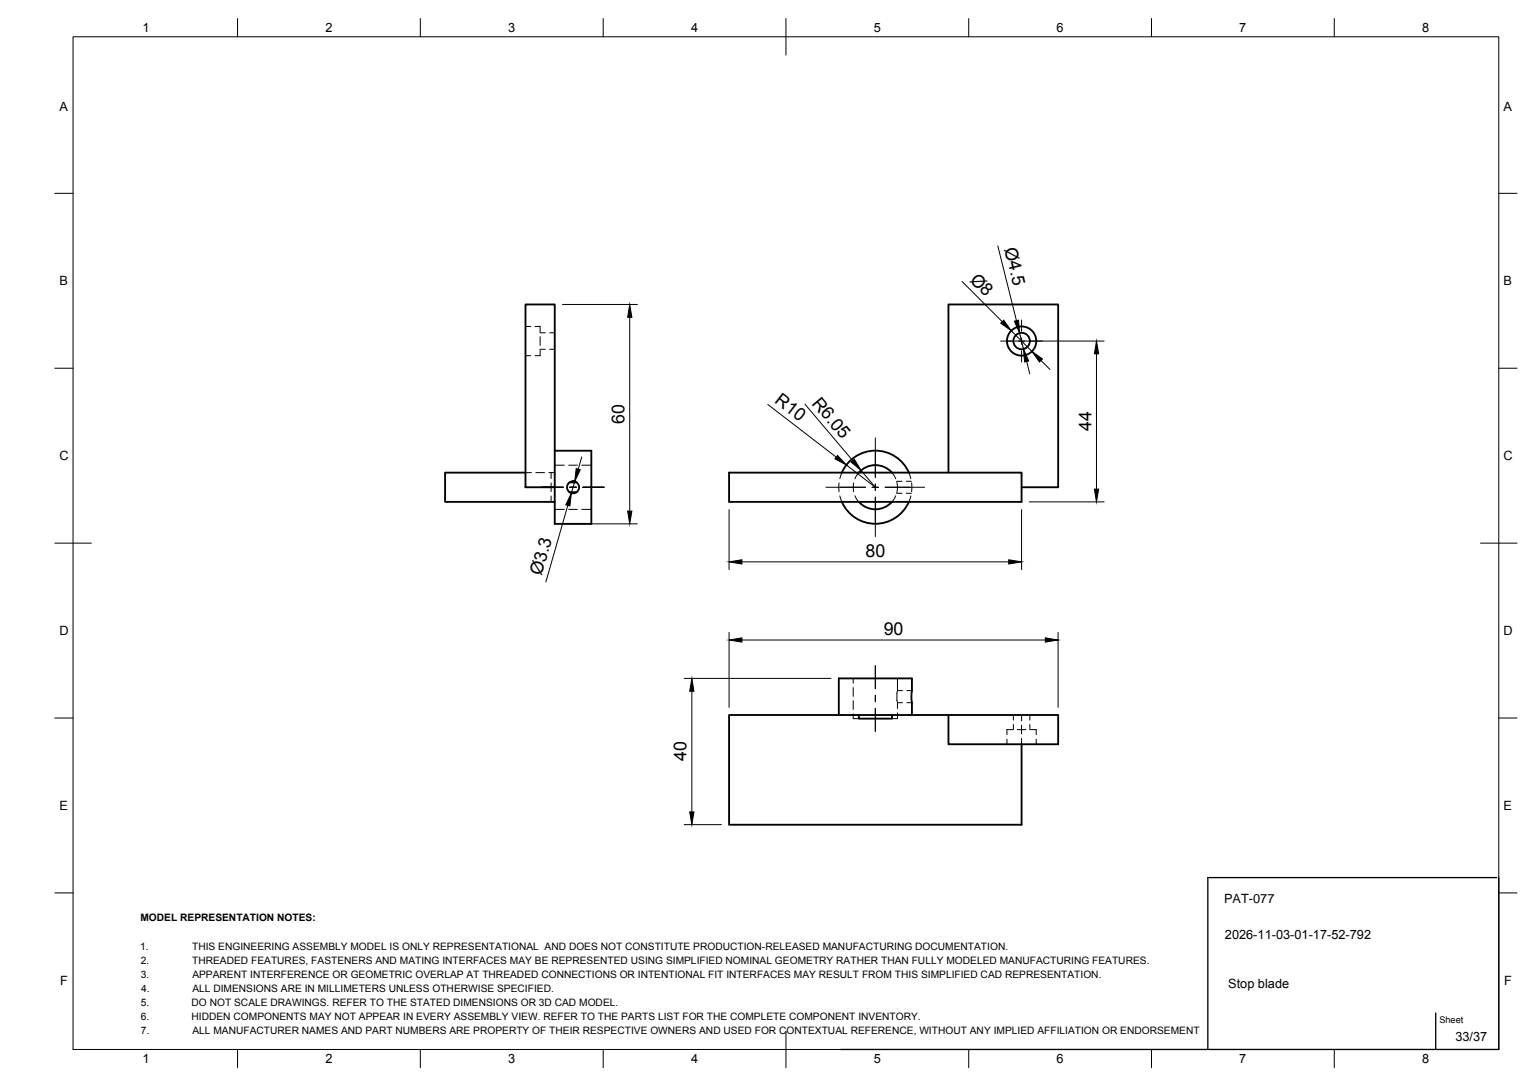
ISO-10303-21;
HEADER;
/* Generated by software containing ST-Developer
 * from STEP Tools, Inc. (www.steptools.com) 
 */

FILE_DESCRIPTION(
/* description */ ('Pallet stop with pneumatic fitting'),
/* implementation_level */ '2;1');

FILE_NAME(
/* name */ 'Stop blade.step',
/* time_stamp */ '2026-10-27T10:51:41-07:00',
/* author */ (''),
/* organization */ (''),
/* preprocessor_version */ 'ST-DEVELOPER v20.2',
/* originating_system */ 'Autodesk Translation Framework v15.17.0.0',
/* authorisation */ '');

FILE_SCHEMA (('AUTOMOTIVE_DESIGN { 1 0 10303 214 3 1 1 }'));
ENDSEC;

DATA;
#10=MECHANICAL_DESIGN_GEOMETRIC_PRESENTATION_REPRESENTATION('',(#382),#10265);
#287=B_SPLINE_CURVE_WITH_KNOTS('',3,(#9812,#9813,#9814,#9815,#9816,#9817,
#9818,#9819,#9820,#9821,#9822,#9823,#9824,#9825),.UNSPECIFIED.,.F.,.F.,
(4,2,2,2,2,2,4),(0.598759573717651,0.624973342427789,0.687463163426141,
0.749952984424493,0.812442805422845,0.874932626421197,0.901146395131335),
 .UNSPECIFIED.);
#288=B_SPLINE_CURVE_WITH_KNOTS('',3,(#9829,#9830,#9831,#9832,#9833,#9834,
#9835,#9836),.UNSPECIFIED.,.F.,.F.,(4,2,2,4),(0.249984328141498,0.31247414913985,
0.374963970138202,0.401177738848337),.UNSPECIFIED.);
#289=B_SPLINE_CURVE_WITH_KNOTS('',3,(#9840,#9841,#9842,#9843,#9844,#9845,
#9846,#9847,#9848,#9849,#9850,#9851,#9852,#9853,#9854,#9855,#9856,#9857,
#9858,#9859,#9860,#9861,#9862,#9863,#9864,#9865),.UNSPECIFIED.,.F.,.F.,
(4,2,2,2,2,2,2,2,2,2,2,2,4),(0.,0.0622766332261793,0.124553266452359,0.186828302721277,
0.249103338990195,0.311378375259114,0.373653411528032,0.435930044754212,
0.498206677980391,0.56048331120657,0.62275994443275,0.685034980701668,0.747310016970586),
 .UNSPECIFIED.);
#290=B_SPLINE_CURVE_WITH_KNOTS('',3,(#9866,#9867,#9868,#9869,#9870,#9871,
#9872,#9873,#9874,#9875),.UNSPECIFIED.,.F.,.F.,(4,2,2,2,4),(0.747310016970586,
0.809585053239505,0.871860089508423,0.934136722734602,0.996413355960782),
 .UNSPECIFIED.);
#291=B_SPLINE_CURVE_WITH_KNOTS('',3,(#9876,#9877,#9878,#9879,#9880,#9881,
#9882,#9883),.UNSPECIFIED.,.F.,.F.,(4,2,2,4),(0.0987909174346565,0.125004686144793,
0.187494507143146,0.249984328141498),.UNSPECIFIED.);
#318=SHAPE_REPRESENTATION_RELATIONSHIP('SRR','None',#10434,#350);
#350=ADVANCED_BREP_SHAPE_REPRESENTATION('',(#413),#10258);
#382=STYLED_ITEM('',(#10641),#413);
#413=MANIFOLD_SOLID_BREP('Body1',#5071);
#529=FACE_BOUND('',#1401,.T.);
#530=FACE_BOUND('',#1408,.T.);
#531=FACE_BOUND('',#1416,.T.);
#532=FACE_BOUND('',#1421,.T.);
#533=FACE_BOUND('',#1423,.T.);
#534=FACE_BOUND('',#1426,.T.);
#685=PLANE('',#5905);
#686=PLANE('',#5909);
#687=PLANE('',#5910);
#688=PLANE('',#5911);
#689=PLANE('',#5912);
#690=PLANE('',#5913);
#691=PLANE('',#5914);
#692=PLANE('',#5915);
#693=PLANE('',#5916);
#694=PLANE('',#5920);
#695=PLANE('',#5921);
#696=PLANE('',#5929);
#697=PLANE('',#5930);
#698=PLANE('',#5932);
#699=PLANE('',#5939);
#700=PLANE('',#5940);
#701=PLANE('',#5941);
#702=PLANE('',#5942);
#703=PLANE('',#5943);
#975=FACE_OUTER_BOUND('',#1399,.T.);
#976=FACE_OUTER_BOUND('',#1400,.T.);
#977=FACE_OUTER_BOUND('',#1402,.T.);
#978=FACE_OUTER_BOUND('',#1403,.T.);
#979=FACE_OUTER_BOUND('',#1404,.T.);
#980=FACE_OUTER_BOUND('',#1405,.T.);
#981=FACE_OUTER_BOUND('',#1406,.T.);
#982=FACE_OUTER_BOUND('',#1407,.T.);
#983=FACE_OUTER_BOUND('',#1409,.T.);
#984=FACE_OUTER_BOUND('',#1410,.T.);
#985=FACE_OUTER_BOUND('',#1411,.T.);
#986=FACE_OUTER_BOUND('',#1412,.T.);
#987=FACE_OUTER_BOUND('',#1413,.T.);
#988=FACE_OUTER_BOUND('',#1414,.T.);
#989=FACE_OUTER_BOUND('',#1415,.T.);
#990=FACE_OUTER_BOUND('',#1417,.T.);
#991=FACE_OUTER_BOUND('',#1418,.T.);
#992=FACE_OUTER_BOUND('',#1419,.T.);
#993=FACE_OUTER_BOUND('',#1420,.T.);
#994=FACE_OUTER_BOUND('',#1422,.T.);
#995=FACE_OUTER_BOUND('',#1424,.T.);
#996=FACE_OUTER_BOUND('',#1425,.T.);
#997=FACE_OUTER_BOUND('',#1427,.T.);
#998=FACE_OUTER_BOUND('',#1428,.T.);
#1399=EDGE_LOOP('',(#4310,#4311,#4312,#4313));
#1400=EDGE_LOOP('',(#4314));
#1401=EDGE_LOOP('',(#4315));
#1402=EDGE_LOOP('',(#4316,#4317,#4318,#4319));
#1403=EDGE_LOOP('',(#4320,#4321,#4322,#4323));
#1404=EDGE_LOOP('',(#4324,#4325,#4326,#4327));
#1405=EDGE_LOOP('',(#4328,#4329,#4330,#4331));
#1406=EDGE_LOOP('',(#4332,#4333,#4334,#4335));
#1407=EDGE_LOOP('',(#4336,#4337,#4338,#4339,#4340,#4341));
#1408=EDGE_LOOP('',(#4342));
#1409=EDGE_LOOP('',(#4343,#4344,#4345,#4346,#4347,#4348));
#1410=EDGE_LOOP('',(#4349,#4350,#4351,#4352,#4353,#4354,#4355,#4356,#4357,
#4358,#4359,#4360));
#1411=EDGE_LOOP('',(#4361,#4362));
#1412=EDGE_LOOP('',(#4363,#4364,#4365,#4366,#4367,#4368,#4369,#4370,#4371));
#1413=EDGE_LOOP('',(#4372,#4373));
#1414=EDGE_LOOP('',(#4374,#4375,#4376,#4377,#4378));
#1415=EDGE_LOOP('',(#4379,#4380,#4381,#4382,#4383,#4384,#4385,#4386,#4387,
#4388,#4389,#4390));
#1416=EDGE_LOOP('',(#4391,#4392,#4393,#4394,#4395));
#1417=EDGE_LOOP('',(#4396,#4397,#4398,#4399,#4400,#4401,#4402,#4403,#4404,
#4405));
#1418=EDGE_LOOP('',(#4406,#4407,#4408,#4409));
#1419=EDGE_LOOP('',(#4410,#4411,#4412,#4413));
#1420=EDGE_LOOP('',(#4414,#4415,#4416,#4417,#4418,#4419,#4420,#4421));
#1421=EDGE_LOOP('',(#4422,#4423));
#1422=EDGE_LOOP('',(#4424));
#1423=EDGE_LOOP('',(#4425));
#1424=EDGE_LOOP('',(#4426,#4427,#4428,#4429,#4430));
#1425=EDGE_LOOP('',(#4431,#4432,#4433,#4434,#4435,#4436,#4437,#4438));
#1426=EDGE_LOOP('',(#4439));
#1427=EDGE_LOOP('',(#4440,#4441,#4442,#4443));
#1428=EDGE_LOOP('',(#4444,#4445,#4446,#4447));
#1724=LINE('',#9739,#2059);
#1725=LINE('',#9747,#2060);
#1726=LINE('',#9751,#2061);
#1727=LINE('',#9753,#2062);
#1728=LINE('',#9755,#2063);
#1729=LINE('',#9756,#2064);
#1730=LINE('',#9759,#2065);
#1731=LINE('',#9761,#2066);
#1732=LINE('',#9762,#2067);
#1733=LINE('',#9765,#2068);
#1734=LINE('',#9767,#2069);
#1735=LINE('',#9768,#2070);
#1736=LINE('',#9772,#2071);
#1737=LINE('',#9773,#2072);
#1738=LINE('',#9774,#2073);
#1739=LINE('',#9777,#2074);
#1740=LINE('',#9778,#2075);
#1741=LINE('',#9781,#2076);
#1742=LINE('',#9783,#2077);
#1743=LINE('',#9785,#2078);
#1744=LINE('',#9786,#2079);
#1745=LINE('',#9789,#2080);
#1746=LINE('',#9791,#2081);
#1747=LINE('',#9793,#2082);
#1748=LINE('',#9795,#2083);
#1749=LINE('',#9797,#2084);
#1750=LINE('',#9799,#2085);
#1751=LINE('',#9801,#2086);
#1752=LINE('',#9803,#2087);
#1753=LINE('',#9804,#2088);
#1754=LINE('',#9808,#2089);
#1755=LINE('',#9838,#2090);
#1756=LINE('',#9885,#2091);
#1757=LINE('',#9890,#2092);
#1758=LINE('',#9897,#2093);
#1759=LINE('',#9899,#2094);
#1760=LINE('',#9902,#2095);
#1761=LINE('',#9906,#2096);
#1762=LINE('',#9907,#2097);
#1763=LINE('',#9909,#2098);
#1764=LINE('',#9911,#2099);
#1765=LINE('',#9913,#2100);
#1766=LINE('',#9914,#2101);
#1767=LINE('',#9925,#2102);
#1768=LINE('',#9929,#2103);
#1769=LINE('',#9932,#2104);
#2059=VECTOR('',#7267,0.4);
#2060=VECTOR('',#7278,0.225);
#2061=VECTOR('',#7281,1.);
#2062=VECTOR('',#7282,1.);
#2063=VECTOR('',#7283,1.);
#2064=VECTOR('',#7284,1.);
#2065=VECTOR('',#7287,1.);
#2066=VECTOR('',#7288,1.);
#2067=VECTOR('',#7289,1.);
#2068=VECTOR('',#7292,1.);
#2069=VECTOR('',#7293,1.);
#2070=VECTOR('',#7294,1.);
#2071=VECTOR('',#7297,1.);
#2072=VECTOR('',#7298,1.);
#2073=VECTOR('',#7299,1.);
#2074=VECTOR('',#7302,1.);
#2075=VECTOR('',#7303,1.);
#2076=VECTOR('',#7306,1.);
#2077=VECTOR('',#7307,1.);
#2078=VECTOR('',#7308,1.);
#2079=VECTOR('',#7309,1.);
#2080=VECTOR('',#7312,1.);
#2081=VECTOR('',#7313,1.);
#2082=VECTOR('',#7314,1.);
#2083=VECTOR('',#7315,1.);
#2084=VECTOR('',#7316,1.);
#2085=VECTOR('',#7317,1.);
#2086=VECTOR('',#7318,1.);
#2087=VECTOR('',#7319,1.);
#2088=VECTOR('',#7320,1.);
#2089=VECTOR('',#7323,1.);
#2090=VECTOR('',#7330,0.164999999999999);
#2091=VECTOR('',#7333,1.);
#2092=VECTOR('',#7338,1.);
#2093=VECTOR('',#7347,0.605);
#2094=VECTOR('',#7348,1.);
#2095=VECTOR('',#7351,1.);
#2096=VECTOR('',#7356,1.);
#2097=VECTOR('',#7357,1.);
#2098=VECTOR('',#7358,1.);
#2099=VECTOR('',#7359,1.);
#2100=VECTOR('',#7360,1.);
#2101=VECTOR('',#7361,1.);
#2102=VECTOR('',#7378,1.);
#2103=VECTOR('',#7385,1.);
#2104=VECTOR('',#7390,1.);
#2357=CIRCLE('',#5903,0.4);
#2358=CIRCLE('',#5904,0.4);
#2359=CIRCLE('',#5906,0.225);
#2360=CIRCLE('',#5908,0.225);
#2361=CIRCLE('',#5917,0.164999999999999);
#2362=CIRCLE('',#5919,0.164999999999999);
#2363=CIRCLE('',#5922,0.605);
#2364=CIRCLE('',#5923,0.605);
#2365=CIRCLE('',#5924,0.605);
#2366=CIRCLE('',#5926,0.605);
#2367=CIRCLE('',#5927,0.605);
#2368=CIRCLE('',#5928,0.605);
#2369=CIRCLE('',#5931,1.);
#2370=CIRCLE('',#5933,1.);
#2371=CIRCLE('',#5935,1.);
#2372=CIRCLE('',#5936,1.);
#2373=CIRCLE('',#5937,1.);
#2374=CIRCLE('',#5938,1.);
#2703=VERTEX_POINT('',#9736);
#2704=VERTEX_POINT('',#9738);
#2705=VERTEX_POINT('',#9742);
#2706=VERTEX_POINT('',#9745);
#2707=VERTEX_POINT('',#9749);
#2708=VERTEX_POINT('',#9750);
#2709=VERTEX_POINT('',#9752);
#2710=VERTEX_POINT('',#9754);
#2711=VERTEX_POINT('',#9758);
#2712=VERTEX_POINT('',#9760);
#2713=VERTEX_POINT('',#9764);
#2714=VERTEX_POINT('',#9766);
#2715=VERTEX_POINT('',#9770);
#2716=VERTEX_POINT('',#9771);
#2717=VERTEX_POINT('',#9776);
#2718=VERTEX_POINT('',#9780);
#2719=VERTEX_POINT('',#9782);
#2720=VERTEX_POINT('',#9784);
#2721=VERTEX_POINT('',#9788);
#2722=VERTEX_POINT('',#9790);
#2723=VERTEX_POINT('',#9792);
#2724=VERTEX_POINT('',#9794);
#2725=VERTEX_POINT('',#9796);
#2726=VERTEX_POINT('',#9798);
#2727=VERTEX_POINT('',#9800);
#2728=VERTEX_POINT('',#9802);
#2729=VERTEX_POINT('',#9806);
#2730=VERTEX_POINT('',#9807);
#2731=VERTEX_POINT('',#9811);
#2732=VERTEX_POINT('',#9826);
#2733=VERTEX_POINT('',#9828);
#2734=VERTEX_POINT('',#9837);
#2735=VERTEX_POINT('',#9839);
#2736=VERTEX_POINT('',#9887);
#2737=VERTEX_POINT('',#9889);
#2738=VERTEX_POINT('',#9891);
#2739=VERTEX_POINT('',#9895);
#2740=VERTEX_POINT('',#9898);
#2741=VERTEX_POINT('',#9900);
#2742=VERTEX_POINT('',#9905);
#2743=VERTEX_POINT('',#9908);
#2744=VERTEX_POINT('',#9910);
#2745=VERTEX_POINT('',#9912);
#2746=VERTEX_POINT('',#9920);
#2747=VERTEX_POINT('',#9924);
#3254=EDGE_CURVE('',#2703,#2703,#2357,.T.);
#3255=EDGE_CURVE('',#2703,#2704,#1724,.T.);
#3256=EDGE_CURVE('',#2704,#2704,#2358,.T.);
#3257=EDGE_CURVE('',#2705,#2705,#2359,.T.);
#3258=EDGE_CURVE('',#2706,#2706,#2360,.T.);
#3259=EDGE_CURVE('',#2706,#2705,#1725,.T.);
#3260=EDGE_CURVE('',#2707,#2708,#1726,.T.);
#3261=EDGE_CURVE('',#2709,#2707,#1727,.T.);
#3262=EDGE_CURVE('',#2710,#2709,#1728,.T.);
#3263=EDGE_CURVE('',#2710,#2708,#1729,.T.);
#3264=EDGE_CURVE('',#2711,#2710,#1730,.T.);
#3265=EDGE_CURVE('',#2712,#2709,#1731,.T.);
#3266=EDGE_CURVE('',#2711,#2712,#1732,.T.);
#3267=EDGE_CURVE('',#2713,#2711,#1733,.T.);
#3268=EDGE_CURVE('',#2714,#2712,#1734,.T.);
#3269=EDGE_CURVE('',#2713,#2714,#1735,.T.);
#3270=EDGE_CURVE('',#2715,#2716,#1736,.T.);
#3271=EDGE_CURVE('',#2715,#2713,#1737,.T.);
#3272=EDGE_CURVE('',#2716,#2714,#1738,.T.);
#3273=EDGE_CURVE('',#2716,#2717,#1739,.T.);
#3274=EDGE_CURVE('',#2717,#2707,#1740,.T.);
#3275=EDGE_CURVE('',#2717,#2718,#1741,.T.);
#3276=EDGE_CURVE('',#2719,#2718,#1742,.T.);
#3277=EDGE_CURVE('',#2720,#2719,#1743,.T.);
#3278=EDGE_CURVE('',#2720,#2715,#1744,.T.);
#3279=EDGE_CURVE('',#2708,#2721,#1745,.T.);
#3280=EDGE_CURVE('',#2721,#2722,#1746,.T.);
#3281=EDGE_CURVE('',#2722,#2723,#1747,.T.);
#3282=EDGE_CURVE('',#2723,#2724,#1748,.T.);
#3283=EDGE_CURVE('',#2724,#2725,#1749,.T.);
#3284=EDGE_CURVE('',#2725,#2726,#1750,.T.);
#3285=EDGE_CURVE('',#2726,#2727,#1751,.T.);
#3286=EDGE_CURVE('',#2727,#2728,#1752,.T.);
#3287=EDGE_CURVE('',#2718,#2728,#1753,.T.);
#3288=EDGE_CURVE('',#2729,#2730,#1754,.T.);
#3289=EDGE_CURVE('',#2729,#2730,#2361,.T.);
#3290=EDGE_CURVE('',#2731,#2729,#287,.T.);
#3291=EDGE_CURVE('',#2732,#2731,#2362,.T.);
#3292=EDGE_CURVE('',#2733,#2732,#288,.T.);
#3293=EDGE_CURVE('',#2733,#2734,#1755,.T.);
#3294=EDGE_CURVE('',#2735,#2734,#289,.T.);
#3295=EDGE_CURVE('',#2734,#2735,#290,.T.);
#3296=EDGE_CURVE('',#2730,#2733,#291,.T.);
#3297=EDGE_CURVE('',#2732,#2731,#1756,.T.);
#3298=EDGE_CURVE('',#2736,#2723,#2363,.T.);
#3299=EDGE_CURVE('',#2737,#2736,#1757,.T.);
#3300=EDGE_CURVE('',#2738,#2737,#2364,.T.);
#3301=EDGE_CURVE('',#2724,#2738,#2365,.T.);
#3302=EDGE_CURVE('',#2739,#2739,#2366,.T.);
#3303=EDGE_CURVE('',#2739,#2738,#1758,.T.);
#3304=EDGE_CURVE('',#2740,#2737,#1759,.T.);
#3305=EDGE_CURVE('',#2741,#2740,#2367,.T.);
#3306=EDGE_CURVE('',#2736,#2741,#1760,.T.);
#3307=EDGE_CURVE('',#2725,#2722,#2368,.T.);
#3308=EDGE_CURVE('',#2741,#2742,#1761,.T.);
#3309=EDGE_CURVE('',#2742,#2720,#1762,.T.);
#3310=EDGE_CURVE('',#2743,#2719,#1763,.T.);
#3311=EDGE_CURVE('',#2744,#2743,#1764,.T.);
#3312=EDGE_CURVE('',#2744,#2745,#1765,.T.);
#3313=EDGE_CURVE('',#2745,#2740,#1766,.T.);
#3314=EDGE_CURVE('',#2721,#2726,#2369,.T.);
#3315=EDGE_CURVE('',#2745,#2742,#2370,.T.);
#3316=EDGE_CURVE('',#2726,#2746,#2371,.T.);
#3317=EDGE_CURVE('',#2742,#2721,#2372,.T.);
#3318=EDGE_CURVE('',#2746,#2745,#2373,.T.);
#3319=EDGE_CURVE('',#2746,#2747,#1767,.T.);
#3320=EDGE_CURVE('',#2747,#2747,#2374,.T.);
#3321=EDGE_CURVE('',#2727,#2744,#1768,.T.);
#3322=EDGE_CURVE('',#2728,#2743,#1769,.T.);
#4310=ORIENTED_EDGE('',*,*,#3254,.F.);
#4311=ORIENTED_EDGE('',*,*,#3255,.T.);
#4312=ORIENTED_EDGE('',*,*,#3256,.F.);
#4313=ORIENTED_EDGE('',*,*,#3255,.F.);
#4314=ORIENTED_EDGE('',*,*,#3254,.T.);
#4315=ORIENTED_EDGE('',*,*,#3257,.F.);
#4316=ORIENTED_EDGE('',*,*,#3258,.F.);
#4317=ORIENTED_EDGE('',*,*,#3259,.T.);
#4318=ORIENTED_EDGE('',*,*,#3257,.T.);
#4319=ORIENTED_EDGE('',*,*,#3259,.F.);
#4320=ORIENTED_EDGE('',*,*,#3260,.F.);
#4321=ORIENTED_EDGE('',*,*,#3261,.F.);
#4322=ORIENTED_EDGE('',*,*,#3262,.F.);
#4323=ORIENTED_EDGE('',*,*,#3263,.T.);
#4324=ORIENTED_EDGE('',*,*,#3264,.T.);
#4325=ORIENTED_EDGE('',*,*,#3262,.T.);
#4326=ORIENTED_EDGE('',*,*,#3265,.F.);
#4327=ORIENTED_EDGE('',*,*,#3266,.F.);
#4328=ORIENTED_EDGE('',*,*,#3267,.T.);
#4329=ORIENTED_EDGE('',*,*,#3266,.T.);
#4330=ORIENTED_EDGE('',*,*,#3268,.F.);
#4331=ORIENTED_EDGE('',*,*,#3269,.F.);
#4332=ORIENTED_EDGE('',*,*,#3270,.F.);
#4333=ORIENTED_EDGE('',*,*,#3271,.T.);
#4334=ORIENTED_EDGE('',*,*,#3269,.T.);
#4335=ORIENTED_EDGE('',*,*,#3272,.F.);
#4336=ORIENTED_EDGE('',*,*,#3273,.F.);
#4337=ORIENTED_EDGE('',*,*,#3272,.T.);
#4338=ORIENTED_EDGE('',*,*,#3268,.T.);
#4339=ORIENTED_EDGE('',*,*,#3265,.T.);
#4340=ORIENTED_EDGE('',*,*,#3261,.T.);
#4341=ORIENTED_EDGE('',*,*,#3274,.F.);
#4342=ORIENTED_EDGE('',*,*,#3256,.T.);
#4343=ORIENTED_EDGE('',*,*,#3270,.T.);
#4344=ORIENTED_EDGE('',*,*,#3273,.T.);
#4345=ORIENTED_EDGE('',*,*,#3275,.T.);
#4346=ORIENTED_EDGE('',*,*,#3276,.F.);
#4347=ORIENTED_EDGE('',*,*,#3277,.F.);
#4348=ORIENTED_EDGE('',*,*,#3278,.T.);
#4349=ORIENTED_EDGE('',*,*,#3274,.T.);
#4350=ORIENTED_EDGE('',*,*,#3260,.T.);
#4351=ORIENTED_EDGE('',*,*,#3279,.T.);
#4352=ORIENTED_EDGE('',*,*,#3280,.T.);
#4353=ORIENTED_EDGE('',*,*,#3281,.T.);
#4354=ORIENTED_EDGE('',*,*,#3282,.T.);
#4355=ORIENTED_EDGE('',*,*,#3283,.T.);
#4356=ORIENTED_EDGE('',*,*,#3284,.T.);
#4357=ORIENTED_EDGE('',*,*,#3285,.T.);
#4358=ORIENTED_EDGE('',*,*,#3286,.T.);
#4359=ORIENTED_EDGE('',*,*,#3287,.F.);
#4360=ORIENTED_EDGE('',*,*,#3275,.F.);
#4361=ORIENTED_EDGE('',*,*,#3288,.F.);
#4362=ORIENTED_EDGE('',*,*,#3289,.T.);
#4363=ORIENTED_EDGE('',*,*,#3290,.F.);
#4364=ORIENTED_EDGE('',*,*,#3291,.F.);
#4365=ORIENTED_EDGE('',*,*,#3292,.F.);
#4366=ORIENTED_EDGE('',*,*,#3293,.T.);
#4367=ORIENTED_EDGE('',*,*,#3294,.F.);
#4368=ORIENTED_EDGE('',*,*,#3295,.F.);
#4369=ORIENTED_EDGE('',*,*,#3293,.F.);
#4370=ORIENTED_EDGE('',*,*,#3296,.F.);
#4371=ORIENTED_EDGE('',*,*,#3289,.F.);
#4372=ORIENTED_EDGE('',*,*,#3297,.F.);
#4373=ORIENTED_EDGE('',*,*,#3291,.T.);
#4374=ORIENTED_EDGE('',*,*,#3282,.F.);
#4375=ORIENTED_EDGE('',*,*,#3298,.F.);
#4376=ORIENTED_EDGE('',*,*,#3299,.F.);
#4377=ORIENTED_EDGE('',*,*,#3300,.F.);
#4378=ORIENTED_EDGE('',*,*,#3301,.F.);
#4379=ORIENTED_EDGE('',*,*,#3302,.F.);
#4380=ORIENTED_EDGE('',*,*,#3303,.T.);
#4381=ORIENTED_EDGE('',*,*,#3300,.T.);
#4382=ORIENTED_EDGE('',*,*,#3304,.F.);
#4383=ORIENTED_EDGE('',*,*,#3305,.F.);
#4384=ORIENTED_EDGE('',*,*,#3306,.F.);
#4385=ORIENTED_EDGE('',*,*,#3298,.T.);
#4386=ORIENTED_EDGE('',*,*,#3281,.F.);
#4387=ORIENTED_EDGE('',*,*,#3307,.F.);
#4388=ORIENTED_EDGE('',*,*,#3283,.F.);
#4389=ORIENTED_EDGE('',*,*,#3301,.T.);
#4390=ORIENTED_EDGE('',*,*,#3303,.F.);
#4391=ORIENTED_EDGE('',*,*,#3296,.T.);
#4392=ORIENTED_EDGE('',*,*,#3292,.T.);
#4393=ORIENTED_EDGE('',*,*,#3297,.T.);
#4394=ORIENTED_EDGE('',*,*,#3290,.T.);
#4395=ORIENTED_EDGE('',*,*,#3288,.T.);
#4396=ORIENTED_EDGE('',*,*,#3304,.T.);
#4397=ORIENTED_EDGE('',*,*,#3299,.T.);
#4398=ORIENTED_EDGE('',*,*,#3306,.T.);
#4399=ORIENTED_EDGE('',*,*,#3308,.T.);
#4400=ORIENTED_EDGE('',*,*,#3309,.T.);
#4401=ORIENTED_EDGE('',*,*,#3277,.T.);
#4402=ORIENTED_EDGE('',*,*,#3310,.F.);
#4403=ORIENTED_EDGE('',*,*,#3311,.F.);
#4404=ORIENTED_EDGE('',*,*,#3312,.T.);
#4405=ORIENTED_EDGE('',*,*,#3313,.T.);
#4406=ORIENTED_EDGE('',*,*,#3307,.T.);
#4407=ORIENTED_EDGE('',*,*,#3280,.F.);
#4408=ORIENTED_EDGE('',*,*,#3314,.T.);
#4409=ORIENTED_EDGE('',*,*,#3284,.F.);
#4410=ORIENTED_EDGE('',*,*,#3305,.T.);
#4411=ORIENTED_EDGE('',*,*,#3313,.F.);
#4412=ORIENTED_EDGE('',*,*,#3315,.T.);
#4413=ORIENTED_EDGE('',*,*,#3308,.F.);
#4414=ORIENTED_EDGE('',*,*,#3316,.F.);
#4415=ORIENTED_EDGE('',*,*,#3314,.F.);
#4416=ORIENTED_EDGE('',*,*,#3317,.F.);
#4417=ORIENTED_EDGE('',*,*,#3315,.F.);
#4418=ORIENTED_EDGE('',*,*,#3318,.F.);
#4419=ORIENTED_EDGE('',*,*,#3319,.T.);
#4420=ORIENTED_EDGE('',*,*,#3320,.T.);
#4421=ORIENTED_EDGE('',*,*,#3319,.F.);
#4422=ORIENTED_EDGE('',*,*,#3294,.T.);
#4423=ORIENTED_EDGE('',*,*,#3295,.T.);
#4424=ORIENTED_EDGE('',*,*,#3320,.F.);
#4425=ORIENTED_EDGE('',*,*,#3302,.T.);
#4426=ORIENTED_EDGE('',*,*,#3316,.T.);
#4427=ORIENTED_EDGE('',*,*,#3318,.T.);
#4428=ORIENTED_EDGE('',*,*,#3312,.F.);
#4429=ORIENTED_EDGE('',*,*,#3321,.F.);
#4430=ORIENTED_EDGE('',*,*,#3285,.F.);
#4431=ORIENTED_EDGE('',*,*,#3278,.F.);
#4432=ORIENTED_EDGE('',*,*,#3309,.F.);
#4433=ORIENTED_EDGE('',*,*,#3317,.T.);
#4434=ORIENTED_EDGE('',*,*,#3279,.F.);
#4435=ORIENTED_EDGE('',*,*,#3263,.F.);
#4436=ORIENTED_EDGE('',*,*,#3264,.F.);
#4437=ORIENTED_EDGE('',*,*,#3267,.F.);
#4438=ORIENTED_EDGE('',*,*,#3271,.F.);
#4439=ORIENTED_EDGE('',*,*,#3258,.T.);
#4440=ORIENTED_EDGE('',*,*,#3321,.T.);
#4441=ORIENTED_EDGE('',*,*,#3311,.T.);
#4442=ORIENTED_EDGE('',*,*,#3322,.F.);
#4443=ORIENTED_EDGE('',*,*,#3286,.F.);
#4444=ORIENTED_EDGE('',*,*,#3322,.T.);
#4445=ORIENTED_EDGE('',*,*,#3310,.T.);
#4446=ORIENTED_EDGE('',*,*,#3276,.T.);
#4447=ORIENTED_EDGE('',*,*,#3287,.T.);
#4713=CYLINDRICAL_SURFACE('',#5902,0.4);
#4714=CYLINDRICAL_SURFACE('',#5907,0.225);
#4715=CYLINDRICAL_SURFACE('',#5918,0.164999999999999);
#4716=CYLINDRICAL_SURFACE('',#5925,0.605);
#4717=CYLINDRICAL_SURFACE('',#5934,1.);
#4970=ADVANCED_FACE('',(#975),#4713,.F.);
#4971=ADVANCED_FACE('',(#976,#529),#685,.T.);
#4972=ADVANCED_FACE('',(#977),#4714,.F.);
#4973=ADVANCED_FACE('',(#978),#686,.T.);
#4974=ADVANCED_FACE('',(#979),#687,.T.);
#4975=ADVANCED_FACE('',(#980),#688,.T.);
#4976=ADVANCED_FACE('',(#981),#689,.T.);
#4977=ADVANCED_FACE('',(#982,#530),#690,.T.);
#4978=ADVANCED_FACE('',(#983),#691,.T.);
#4979=ADVANCED_FACE('',(#984),#692,.T.);
#4980=ADVANCED_FACE('',(#985),#693,.T.);
#4981=ADVANCED_FACE('',(#986),#4715,.F.);
#4982=ADVANCED_FACE('',(#987),#694,.T.);
#4983=ADVANCED_FACE('',(#988),#695,.F.);
#4984=ADVANCED_FACE('',(#989,#531),#4716,.F.);
#4985=ADVANCED_FACE('',(#990),#696,.T.);
#4986=ADVANCED_FACE('',(#991),#697,.T.);
#4987=ADVANCED_FACE('',(#992),#698,.T.);
#4988=ADVANCED_FACE('',(#993,#532),#4717,.T.);
#4989=ADVANCED_FACE('',(#994,#533),#699,.F.);
#4990=ADVANCED_FACE('',(#995),#700,.F.);
#4991=ADVANCED_FACE('',(#996,#534),#701,.F.);
#4992=ADVANCED_FACE('',(#997),#702,.T.);
#4993=ADVANCED_FACE('',(#998),#703,.T.);
#5071=CLOSED_SHELL('',(#4970,#4971,#4972,#4973,#4974,#4975,#4976,#4977,
#4978,#4979,#4980,#4981,#4982,#4983,#4984,#4985,#4986,#4987,#4988,#4989,
#4990,#4991,#4992,#4993));
#5901=AXIS2_PLACEMENT_3D('',#9734,#7261,#7262);
#5902=AXIS2_PLACEMENT_3D('',#9735,#7263,#7264);
#5903=AXIS2_PLACEMENT_3D('',#9737,#7265,#7266);
#5904=AXIS2_PLACEMENT_3D('',#9740,#7268,#7269);
#5905=AXIS2_PLACEMENT_3D('',#9741,#7270,#7271);
#5906=AXIS2_PLACEMENT_3D('',#9743,#7272,#7273);
#5907=AXIS2_PLACEMENT_3D('',#9744,#7274,#7275);
#5908=AXIS2_PLACEMENT_3D('',#9746,#7276,#7277);
#5909=AXIS2_PLACEMENT_3D('',#9748,#7279,#7280);
#5910=AXIS2_PLACEMENT_3D('',#9757,#7285,#7286);
#5911=AXIS2_PLACEMENT_3D('',#9763,#7290,#7291);
#5912=AXIS2_PLACEMENT_3D('',#9769,#7295,#7296);
#5913=AXIS2_PLACEMENT_3D('',#9775,#7300,#7301);
#5914=AXIS2_PLACEMENT_3D('',#9779,#7304,#7305);
#5915=AXIS2_PLACEMENT_3D('',#9787,#7310,#7311);
#5916=AXIS2_PLACEMENT_3D('',#9805,#7321,#7322);
#5917=AXIS2_PLACEMENT_3D('',#9809,#7324,#7325);
#5918=AXIS2_PLACEMENT_3D('',#9810,#7326,#7327);
#5919=AXIS2_PLACEMENT_3D('',#9827,#7328,#7329);
#5920=AXIS2_PLACEMENT_3D('',#9884,#7331,#7332);
#5921=AXIS2_PLACEMENT_3D('',#9886,#7334,#7335);
#5922=AXIS2_PLACEMENT_3D('',#9888,#7336,#7337);
#5923=AXIS2_PLACEMENT_3D('',#9892,#7339,#7340);
#5924=AXIS2_PLACEMENT_3D('',#9893,#7341,#7342);
#5925=AXIS2_PLACEMENT_3D('',#9894,#7343,#7344);
#5926=AXIS2_PLACEMENT_3D('',#9896,#7345,#7346);
#5927=AXIS2_PLACEMENT_3D('',#9901,#7349,#7350);
#5928=AXIS2_PLACEMENT_3D('',#9903,#7352,#7353);
#5929=AXIS2_PLACEMENT_3D('',#9904,#7354,#7355);
#5930=AXIS2_PLACEMENT_3D('',#9915,#7362,#7363);
#5931=AXIS2_PLACEMENT_3D('',#9916,#7364,#7365);
#5932=AXIS2_PLACEMENT_3D('',#9917,#7366,#7367);
#5933=AXIS2_PLACEMENT_3D('',#9918,#7368,#7369);
#5934=AXIS2_PLACEMENT_3D('',#9919,#7370,#7371);
#5935=AXIS2_PLACEMENT_3D('',#9921,#7372,#7373);
#5936=AXIS2_PLACEMENT_3D('',#9922,#7374,#7375);
#5937=AXIS2_PLACEMENT_3D('',#9923,#7376,#7377);
#5938=AXIS2_PLACEMENT_3D('',#9926,#7379,#7380);
#5939=AXIS2_PLACEMENT_3D('',#9927,#7381,#7382);
#5940=AXIS2_PLACEMENT_3D('',#9928,#7383,#7384);
#5941=AXIS2_PLACEMENT_3D('',#9930,#7386,#7387);
#5942=AXIS2_PLACEMENT_3D('',#9931,#7388,#7389);
#5943=AXIS2_PLACEMENT_3D('',#9933,#7391,#7392);
#7261=DIRECTION('axis',(0.,0.,1.));
#7262=DIRECTION('refdir',(1.,0.,0.));
#7263=DIRECTION('center_axis',(0.,0.,1.));
#7264=DIRECTION('ref_axis',(1.,0.,0.));
#7265=DIRECTION('center_axis',(0.,0.,1.));
#7266=DIRECTION('ref_axis',(1.,0.,0.));
#7267=DIRECTION('',(0.,0.,1.));
#7268=DIRECTION('center_axis',(0.,0.,-1.));
#7269=DIRECTION('ref_axis',(1.,0.,0.));
#7270=DIRECTION('center_axis',(0.,0.,1.));
#7271=DIRECTION('ref_axis',(1.,0.,0.));
#7272=DIRECTION('center_axis',(0.,0.,1.));
#7273=DIRECTION('ref_axis',(1.,0.,0.));
#7274=DIRECTION('center_axis',(0.,0.,1.));
#7275=DIRECTION('ref_axis',(1.,0.,0.));
#7276=DIRECTION('center_axis',(0.,0.,1.));
#7277=DIRECTION('ref_axis',(1.,0.,0.));
#7278=DIRECTION('',(0.,0.,1.));
#7279=DIRECTION('center_axis',(-1.,0.,0.));
#7280=DIRECTION('ref_axis',(0.,-1.,0.));
#7281=DIRECTION('',(0.,0.,-1.));
#7282=DIRECTION('',(0.,-1.,0.));
#7283=DIRECTION('',(0.,0.,1.));
#7284=DIRECTION('',(0.,-1.,0.));
#7285=DIRECTION('center_axis',(0.,1.,0.));
#7286=DIRECTION('ref_axis',(-1.,0.,0.));
#7287=DIRECTION('',(-1.,0.,0.));
#7288=DIRECTION('',(-1.,0.,0.));
#7289=DIRECTION('',(0.,0.,1.));
#7290=DIRECTION('center_axis',(1.,0.,0.));
#7291=DIRECTION('ref_axis',(0.,1.,0.));
#7292=DIRECTION('',(0.,1.,0.));
#7293=DIRECTION('',(0.,1.,0.));
#7294=DIRECTION('',(0.,0.,1.));
#7295=DIRECTION('center_axis',(0.,-1.,0.));
#7296=DIRECTION('ref_axis',(1.,0.,0.));
#7297=DIRECTION('',(0.,0.,1.));
#7298=DIRECTION('',(1.,0.,0.));
#7299=DIRECTION('',(1.,0.,0.));
#7300=DIRECTION('center_axis',(0.,0.,1.));
#7301=DIRECTION('ref_axis',(1.,0.,0.));
#7302=DIRECTION('',(0.,1.,0.));
#7303=DIRECTION('',(-1.,0.,0.));
#7304=DIRECTION('center_axis',(1.,0.,0.));
#7305=DIRECTION('ref_axis',(0.,1.,0.));
#7306=DIRECTION('',(0.,0.,1.));
#7307=DIRECTION('',(0.,1.,0.));
#7308=DIRECTION('',(0.,0.,1.));
#7309=DIRECTION('',(0.,1.,0.));
#7310=DIRECTION('center_axis',(0.,1.,0.));
#7311=DIRECTION('ref_axis',(-1.,0.,0.));
#7312=DIRECTION('',(-1.,0.,0.));
#7313=DIRECTION('',(-1.,0.,0.));
#7314=DIRECTION('',(0.,0.,1.));
#7315=DIRECTION('',(-1.,0.,0.));
#7316=DIRECTION('',(0.,0.,-1.));
#7317=DIRECTION('',(-1.,0.,0.));
#7318=DIRECTION('',(-1.,0.,0.));
#7319=DIRECTION('',(0.,0.,1.));
#7320=DIRECTION('',(-1.,0.,0.));
#7321=DIRECTION('center_axis',(1.,0.,0.));
#7322=DIRECTION('ref_axis',(0.,0.,-1.));
#7323=DIRECTION('',(0.,0.,1.));
#7324=DIRECTION('center_axis',(1.,0.,0.));
#7325=DIRECTION('ref_axis',(0.,0.,-1.));
#7326=DIRECTION('center_axis',(1.,0.,0.));
#7327=DIRECTION('ref_axis',(0.,0.,-1.));
#7328=DIRECTION('center_axis',(1.,0.,0.));
#7329=DIRECTION('ref_axis',(0.,0.,-1.));
#7330=DIRECTION('',(1.,0.,0.));
#7331=DIRECTION('center_axis',(1.,0.,0.));
#7332=DIRECTION('ref_axis',(0.,0.,-1.));
#7333=DIRECTION('',(0.,0.,-1.));
#7334=DIRECTION('center_axis',(0.,0.,1.));
#7335=DIRECTION('ref_axis',(1.,0.,0.));
#7336=DIRECTION('center_axis',(0.,0.,1.));
#7337=DIRECTION('ref_axis',(1.,0.,0.));
#7338=DIRECTION('',(1.,0.,0.));
#7339=DIRECTION('center_axis',(0.,0.,1.));
#7340=DIRECTION('ref_axis',(1.,0.,0.));
#7341=DIRECTION('center_axis',(0.,0.,1.));
#7342=DIRECTION('ref_axis',(1.,0.,0.));
#7343=DIRECTION('center_axis',(0.,0.,1.));
#7344=DIRECTION('ref_axis',(1.,0.,0.));
#7345=DIRECTION('center_axis',(0.,0.,1.));
#7346=DIRECTION('ref_axis',(1.,0.,0.));
#7347=DIRECTION('',(0.,0.,1.));
#7348=DIRECTION('',(0.,0.,1.));
#7349=DIRECTION('center_axis',(0.,0.,-1.));
#7350=DIRECTION('ref_axis',(1.,0.,0.));
#7351=DIRECTION('',(0.,0.,-1.));
#7352=DIRECTION('center_axis',(0.,0.,-1.));
#7353=DIRECTION('ref_axis',(1.,0.,0.));
#7354=DIRECTION('center_axis',(0.,-1.,0.));
#7355=DIRECTION('ref_axis',(1.,0.,0.));
#7356=DIRECTION('',(1.,0.,0.));
#7357=DIRECTION('',(1.,0.,0.));
#7358=DIRECTION('',(1.,0.,0.));
#7359=DIRECTION('',(0.,0.,1.));
#7360=DIRECTION('',(1.,0.,0.));
#7361=DIRECTION('',(1.,0.,0.));
#7362=DIRECTION('center_axis',(0.,0.,1.));
#7363=DIRECTION('ref_axis',(1.,0.,0.));
#7364=DIRECTION('center_axis',(0.,0.,1.));
#7365=DIRECTION('ref_axis',(1.,0.,0.));
#7366=DIRECTION('center_axis',(0.,0.,1.));
#7367=DIRECTION('ref_axis',(1.,0.,0.));
#7368=DIRECTION('center_axis',(0.,0.,1.));
#7369=DIRECTION('ref_axis',(1.,0.,0.));
#7370=DIRECTION('center_axis',(0.,0.,1.));
#7371=DIRECTION('ref_axis',(1.,0.,0.));
#7372=DIRECTION('center_axis',(0.,0.,1.));
#7373=DIRECTION('ref_axis',(1.,0.,0.));
#7374=DIRECTION('center_axis',(0.,0.,1.));
#7375=DIRECTION('ref_axis',(1.,0.,0.));
#7376=DIRECTION('center_axis',(0.,0.,1.));
#7377=DIRECTION('ref_axis',(1.,0.,0.));
#7378=DIRECTION('',(0.,0.,-1.));
#7379=DIRECTION('center_axis',(0.,0.,1.));
#7380=DIRECTION('ref_axis',(1.,0.,0.));
#7381=DIRECTION('center_axis',(0.,0.,1.));
#7382=DIRECTION('ref_axis',(1.,0.,0.));
#7383=DIRECTION('center_axis',(0.,0.,1.));
#7384=DIRECTION('ref_axis',(1.,0.,0.));
#7385=DIRECTION('',(0.,-1.,0.));
#7386=DIRECTION('center_axis',(0.,0.,1.));
#7387=DIRECTION('ref_axis',(1.,0.,0.));
#7388=DIRECTION('center_axis',(-1.,0.,0.));
#7389=DIRECTION('ref_axis',(0.,-1.,0.));
#7390=DIRECTION('',(0.,-1.,0.));
#7391=DIRECTION('center_axis',(0.,0.,1.));
#7392=DIRECTION('ref_axis',(1.,0.,0.));
#9734=CARTESIAN_POINT('',(0.,0.,0.));
#9735=CARTESIAN_POINT('Origin',(4.,4.,13.4));
#9736=CARTESIAN_POINT('',(3.6,4.,13.4));
#9737=CARTESIAN_POINT('Origin',(4.,4.,13.4));
#9738=CARTESIAN_POINT('',(3.6,4.,13.8));
#9739=CARTESIAN_POINT('',(3.6,4.,13.4));
#9740=CARTESIAN_POINT('Origin',(4.,4.,13.8));
#9741=CARTESIAN_POINT('Origin',(4.,4.,13.4));
#9742=CARTESIAN_POINT('',(3.775,4.,13.4));
#9743=CARTESIAN_POINT('Origin',(4.,4.,13.4));
#9744=CARTESIAN_POINT('Origin',(4.,4.,12.9));
#9745=CARTESIAN_POINT('',(3.775,4.,13.));
#9746=CARTESIAN_POINT('Origin',(4.,4.,13.));
#9747=CARTESIAN_POINT('',(3.775,4.,12.9));
#9748=CARTESIAN_POINT('Origin',(2.,5.,13.));
#9749=CARTESIAN_POINT('',(2.,0.4,13.8));
#9750=CARTESIAN_POINT('',(2.,0.4,13.));
#9751=CARTESIAN_POINT('',(2.,0.4,13.));
#9752=CARTESIAN_POINT('',(2.,5.,13.8));
#9753=CARTESIAN_POINT('',(2.,5.,13.8));
#9754=CARTESIAN_POINT('',(2.,5.,13.));
#9755=CARTESIAN_POINT('',(2.,5.,13.));
#9756=CARTESIAN_POINT('',(2.,5.,13.));
#9757=CARTESIAN_POINT('Origin',(5.,5.,13.));
#9758=CARTESIAN_POINT('',(5.,5.,13.));
#9759=CARTESIAN_POINT('',(5.,5.,13.));
#9760=CARTESIAN_POINT('',(5.,5.,13.8));
#9761=CARTESIAN_POINT('',(5.,5.,13.8));
#9762=CARTESIAN_POINT('',(5.,5.,13.));
#9763=CARTESIAN_POINT('Origin',(5.,0.,13.));
#9764=CARTESIAN_POINT('',(5.,0.,13.));
#9765=CARTESIAN_POINT('',(5.,0.,13.));
#9766=CARTESIAN_POINT('',(5.,0.,13.8));
#9767=CARTESIAN_POINT('',(5.,0.,13.8));
#9768=CARTESIAN_POINT('',(5.,0.,13.));
#9769=CARTESIAN_POINT('Origin',(2.,0.,13.));
#9770=CARTESIAN_POINT('',(4.,0.,13.));
#9771=CARTESIAN_POINT('',(4.,0.,13.8));
#9772=CARTESIAN_POINT('',(4.,0.,13.));
#9773=CARTESIAN_POINT('',(2.,0.,13.));
#9774=CARTESIAN_POINT('',(2.,0.,13.8));
#9775=CARTESIAN_POINT('Origin',(3.5,2.5,13.8));
#9776=CARTESIAN_POINT('',(4.,0.4,13.8));
#9777=CARTESIAN_POINT('',(4.,1.05,13.8));
#9778=CARTESIAN_POINT('',(3.75,0.4,13.8));
#9779=CARTESIAN_POINT('Origin',(4.,-0.4,13.));
#9780=CARTESIAN_POINT('',(4.,0.4,16.));
#9781=CARTESIAN_POINT('',(4.,0.4,13.));
#9782=CARTESIAN_POINT('',(4.,-0.4,16.));
#9783=CARTESIAN_POINT('',(4.,-0.4,16.));
#9784=CARTESIAN_POINT('',(4.,-0.4,13.));
#9785=CARTESIAN_POINT('',(4.,-0.4,13.));
#9786=CARTESIAN_POINT('',(4.,-0.4,13.));
#9787=CARTESIAN_POINT('Origin',(4.,0.4,13.));
#9788=CARTESIAN_POINT('',(0.916515138991168,0.4,13.));
#9789=CARTESIAN_POINT('',(4.,0.4,13.));
#9790=CARTESIAN_POINT('',(0.453899768671455,0.4,13.));
#9791=CARTESIAN_POINT('',(4.,0.4,13.));
#9792=CARTESIAN_POINT('',(0.453899768671455,0.4,13.1));
#9793=CARTESIAN_POINT('',(0.453899768671455,0.4,11.9));
#9794=CARTESIAN_POINT('',(-0.453899768671455,0.4,13.1));
#9795=CARTESIAN_POINT('',(2.,0.4,13.1));
#9796=CARTESIAN_POINT('',(-0.453899768671455,0.4,13.));
#9797=CARTESIAN_POINT('',(-0.453899768671455,0.4,11.9));
#9798=CARTESIAN_POINT('',(-0.916515138991168,0.4,13.));
#9799=CARTESIAN_POINT('',(4.,0.4,13.));
#9800=CARTESIAN_POINT('',(-4.,0.4,13.));
#9801=CARTESIAN_POINT('',(4.,0.4,13.));
#9802=CARTESIAN_POINT('',(-4.,0.4,16.));
#9803=CARTESIAN_POINT('',(-4.,0.4,13.));
#9804=CARTESIAN_POINT('',(4.,0.4,16.));
#9805=CARTESIAN_POINT('Origin',(0.59,0.,12.5));
#9806=CARTESIAN_POINT('',(0.59,0.133884278389959,12.4035634923901));
#9807=CARTESIAN_POINT('',(0.59,0.133884278389959,12.5964365076099));
#9808=CARTESIAN_POINT('',(0.59,0.133884278389959,11.9));
#9809=CARTESIAN_POINT('Origin',(0.59,0.,12.5));
#9810=CARTESIAN_POINT('Origin',(0.59,0.,12.5));
#9811=CARTESIAN_POINT('',(0.59,-0.133884278389959,12.4035634923901));
#9812=CARTESIAN_POINT('Ctrl Pts',(0.59,-0.133884278389958,12.4035634923901));
#9813=CARTESIAN_POINT('Ctrl Pts',(0.591198403406107,-0.128603165341392,
12.3962316423768));
#9814=CARTESIAN_POINT('Ctrl Pts',(0.59244064128815,-0.122792448979943,12.3894472111884));
#9815=CARTESIAN_POINT('Ctrl Pts',(0.596510641114135,-0.10208383195986,12.3687385941683));
#9816=CARTESIAN_POINT('Ctrl Pts',(0.599544094983168,-0.0836002135946602,
12.3560565239921));
#9817=CARTESIAN_POINT('Ctrl Pts',(0.603817074382983,-0.0429774150042656,
12.3391843843662));
#9818=CARTESIAN_POINT('Ctrl Pts',(0.605,-0.0208299403327841,12.335));
#9819=CARTESIAN_POINT('Ctrl Pts',(0.605,0.020829940332784,12.335));
#9820=CARTESIAN_POINT('Ctrl Pts',(0.603817074382983,0.0429774150042655,
12.3391843843662));
#9821=CARTESIAN_POINT('Ctrl Pts',(0.599544094983168,0.0836002135946602,
12.3560565239921));
#9822=CARTESIAN_POINT('Ctrl Pts',(0.596510641114135,0.10208383195986,12.3687385941683));
#9823=CARTESIAN_POINT('Ctrl Pts',(0.59244064128815,0.122792448979943,12.3894472111884));
#9824=CARTESIAN_POINT('Ctrl Pts',(0.591198403406107,0.128603165341392,12.3962316423768));
#9825=CARTESIAN_POINT('Ctrl Pts',(0.59,0.133884278389958,12.4035634923901));
#9826=CARTESIAN_POINT('',(0.59,-0.133884278389959,12.5964365076099));
#9827=CARTESIAN_POINT('Origin',(0.59,0.,12.5));
#9828=CARTESIAN_POINT('',(0.605,3.67341977584082E-17,12.665));
#9829=CARTESIAN_POINT('Ctrl Pts',(0.605,7.63278329429795E-17,12.665));
#9830=CARTESIAN_POINT('Ctrl Pts',(0.605,-0.020829940332784,12.665));
#9831=CARTESIAN_POINT('Ctrl Pts',(0.603817074382983,-0.0429774150042655,
12.6608156156338));
#9832=CARTESIAN_POINT('Ctrl Pts',(0.599544094983168,-0.0836002135946602,
12.6439434760079));
#9833=CARTESIAN_POINT('Ctrl Pts',(0.596510641114135,-0.10208383195986,12.6312614058317));
#9834=CARTESIAN_POINT('Ctrl Pts',(0.59244064128815,-0.122792448979942,12.6105527888116));
#9835=CARTESIAN_POINT('Ctrl Pts',(0.591198403406107,-0.128603165341392,
12.6037683576232));
#9836=CARTESIAN_POINT('Ctrl Pts',(0.59,-0.133884278389959,12.5964365076099));
#9837=CARTESIAN_POINT('',(1.,-2.02066721859312E-17,12.665));
#9838=CARTESIAN_POINT('',(0.59,-2.02066721859312E-17,12.665));
#9839=CARTESIAN_POINT('',(0.986293566845085,0.164999999999999,12.5));
#9840=CARTESIAN_POINT('Ctrl Pts',(0.986293566845085,0.164999999999999,12.5));
#9841=CARTESIAN_POINT('Ctrl Pts',(0.986293566845085,0.164999999999999,12.4792411222579));
#9842=CARTESIAN_POINT('Ctrl Pts',(0.987016731044511,0.160843546393744,12.4571250491954));
#9843=CARTESIAN_POINT('Ctrl Pts',(0.989615421633511,0.143993021293681,12.4164840215393));
#9844=CARTESIAN_POINT('Ctrl Pts',(0.991451962924594,0.131300979727688,12.3979557419361));
#9845=CARTESIAN_POINT('Ctrl Pts',(0.994888849961666,0.102044633178354,12.3686993953868));
#9846=CARTESIAN_POINT('Ctrl Pts',(0.996714420415386,0.0835161924492572,
12.3560070595837));
#9847=CARTESIAN_POINT('Ctrl Pts',(0.99928792543863,0.0428746115883117,12.3391563208071));
#9848=CARTESIAN_POINT('Ctrl Pts',(1.,0.0207583454229728,12.335));
#9849=CARTESIAN_POINT('Ctrl Pts',(1.,-0.0207583454229728,12.335));
#9850=CARTESIAN_POINT('Ctrl Pts',(0.99928792543863,-0.0428746115883117,
12.3391563208071));
#9851=CARTESIAN_POINT('Ctrl Pts',(0.996714420415386,-0.0835161924492572,
12.3560070595837));
#9852=CARTESIAN_POINT('Ctrl Pts',(0.994888849961666,-0.102044633178354,
12.3686993953868));
#9853=CARTESIAN_POINT('Ctrl Pts',(0.991451962924594,-0.131300979727688,
12.3979557419361));
#9854=CARTESIAN_POINT('Ctrl Pts',(0.989615421633511,-0.143993021293681,
12.4164840215393));
#9855=CARTESIAN_POINT('Ctrl Pts',(0.987016731044511,-0.160843546393744,
12.4571250491954));
#9856=CARTESIAN_POINT('Ctrl Pts',(0.986293566845085,-0.164999999999999,
12.4792411222579));
#9857=CARTESIAN_POINT('Ctrl Pts',(0.986293566845085,-0.164999999999999,
12.5207588777421));
#9858=CARTESIAN_POINT('Ctrl Pts',(0.987016731044511,-0.160843546393744,
12.5428749508046));
#9859=CARTESIAN_POINT('Ctrl Pts',(0.989615421633511,-0.143993021293681,
12.5835159784607));
#9860=CARTESIAN_POINT('Ctrl Pts',(0.991451962924594,-0.131300979727688,
12.6020442580639));
#9861=CARTESIAN_POINT('Ctrl Pts',(0.994888849961666,-0.102044633178354,
12.6313006046132));
#9862=CARTESIAN_POINT('Ctrl Pts',(0.996714420415386,-0.0835161924492572,
12.6439929404163));
#9863=CARTESIAN_POINT('Ctrl Pts',(0.99928792543863,-0.0428746115883117,
12.6608436791929));
#9864=CARTESIAN_POINT('Ctrl Pts',(1.,-0.0207583454229728,12.665));
#9865=CARTESIAN_POINT('Ctrl Pts',(1.,-4.85722573273506E-17,12.665));
#9866=CARTESIAN_POINT('Ctrl Pts',(1.,-9.36750677027476E-17,12.665));
#9867=CARTESIAN_POINT('Ctrl Pts',(1.,0.0207583454229727,12.665));
#9868=CARTESIAN_POINT('Ctrl Pts',(0.99928792543863,0.0428746115883117,12.6608436791929));
#9869=CARTESIAN_POINT('Ctrl Pts',(0.996714420415386,0.0835161924492572,
12.6439929404163));
#9870=CARTESIAN_POINT('Ctrl Pts',(0.994888849961666,0.102044633178354,12.6313006046132));
#9871=CARTESIAN_POINT('Ctrl Pts',(0.991451962924594,0.131300979727688,12.6020442580639));
#9872=CARTESIAN_POINT('Ctrl Pts',(0.989615421633511,0.143993021293681,12.5835159784607));
#9873=CARTESIAN_POINT('Ctrl Pts',(0.987016731044511,0.160843546393744,12.5428749508046));
#9874=CARTESIAN_POINT('Ctrl Pts',(0.986293566845085,0.164999999999999,12.5207588777421));
#9875=CARTESIAN_POINT('Ctrl Pts',(0.986293566845085,0.164999999999999,12.5));
#9876=CARTESIAN_POINT('Ctrl Pts',(0.59,0.133884278389959,12.5964365076099));
#9877=CARTESIAN_POINT('Ctrl Pts',(0.591198403406107,0.128603165341392,12.6037683576232));
#9878=CARTESIAN_POINT('Ctrl Pts',(0.59244064128815,0.122792448979943,12.6105527888116));
#9879=CARTESIAN_POINT('Ctrl Pts',(0.596510641114135,0.10208383195986,12.6312614058317));
#9880=CARTESIAN_POINT('Ctrl Pts',(0.599544094983168,0.0836002135946602,
12.6439434760079));
#9881=CARTESIAN_POINT('Ctrl Pts',(0.603817074382983,0.0429774150042655,
12.6608156156338));
#9882=CARTESIAN_POINT('Ctrl Pts',(0.605,0.020829940332784,12.665));
#9883=CARTESIAN_POINT('Ctrl Pts',(0.605,-2.77555756156289E-17,12.665));
#9884=CARTESIAN_POINT('Origin',(0.59,0.,12.5));
#9885=CARTESIAN_POINT('',(0.59,-0.133884278389959,11.9));
#9886=CARTESIAN_POINT('Origin',(0.,0.,13.1));
#9887=CARTESIAN_POINT('',(0.453899768671455,-0.4,13.1));
#9888=CARTESIAN_POINT('Origin',(0.,0.,13.1));
#9889=CARTESIAN_POINT('',(-0.453899768671455,-0.4,13.1));
#9890=CARTESIAN_POINT('',(-2.,-0.4,13.1));
#9891=CARTESIAN_POINT('',(-0.605,-7.40911313484149E-17,13.1));
#9892=CARTESIAN_POINT('Origin',(0.,0.,13.1));
#9893=CARTESIAN_POINT('Origin',(0.,0.,13.1));
#9894=CARTESIAN_POINT('Origin',(0.,0.,11.9));
#9895=CARTESIAN_POINT('',(-0.605,-7.40911313484149E-17,12.));
#9896=CARTESIAN_POINT('Origin',(0.,0.,12.));
#9897=CARTESIAN_POINT('',(-0.605,-7.40911313484149E-17,11.9));
#9898=CARTESIAN_POINT('',(-0.453899768671455,-0.4,13.));
#9899=CARTESIAN_POINT('',(-0.453899768671455,-0.4,11.9));
#9900=CARTESIAN_POINT('',(0.453899768671455,-0.4,13.));
#9901=CARTESIAN_POINT('Origin',(0.,0.,13.));
#9902=CARTESIAN_POINT('',(0.453899768671455,-0.4,11.9));
#9903=CARTESIAN_POINT('Origin',(0.,0.,13.));
#9904=CARTESIAN_POINT('Origin',(-4.,-0.4,13.));
#9905=CARTESIAN_POINT('',(0.916515138991168,-0.4,13.));
#9906=CARTESIAN_POINT('',(-4.,-0.4,13.));
#9907=CARTESIAN_POINT('',(-4.,-0.4,13.));
#9908=CARTESIAN_POINT('',(-4.,-0.4,16.));
#9909=CARTESIAN_POINT('',(-4.,-0.4,16.));
#9910=CARTESIAN_POINT('',(-4.,-0.4,13.));
#9911=CARTESIAN_POINT('',(-4.,-0.4,13.));
#9912=CARTESIAN_POINT('',(-0.916515138991168,-0.4,13.));
#9913=CARTESIAN_POINT('',(-4.,-0.4,13.));
#9914=CARTESIAN_POINT('',(-4.,-0.4,13.));
#9915=CARTESIAN_POINT('Origin',(0.,0.,13.));
#9916=CARTESIAN_POINT('Origin',(0.,0.,13.));
#9917=CARTESIAN_POINT('Origin',(0.,0.,13.));
#9918=CARTESIAN_POINT('Origin',(0.,0.,13.));
#9919=CARTESIAN_POINT('Origin',(0.,0.,12.));
#9920=CARTESIAN_POINT('',(-1.,-1.22464679914735E-16,13.));
#9921=CARTESIAN_POINT('Origin',(0.,0.,13.));
#9922=CARTESIAN_POINT('Origin',(0.,0.,13.));
#9923=CARTESIAN_POINT('Origin',(0.,0.,13.));
#9924=CARTESIAN_POINT('',(-1.,-1.22464679914735E-16,12.));
#9925=CARTESIAN_POINT('',(-1.,-1.22464679914735E-16,12.));
#9926=CARTESIAN_POINT('Origin',(0.,0.,12.));
#9927=CARTESIAN_POINT('Origin',(0.,0.,12.));
#9928=CARTESIAN_POINT('Origin',(0.,0.,13.));
#9929=CARTESIAN_POINT('',(-4.,0.4,13.));
#9930=CARTESIAN_POINT('Origin',(0.,0.,13.));
#9931=CARTESIAN_POINT('Origin',(-4.,0.4,13.));
#9932=CARTESIAN_POINT('',(-4.,0.4,16.));
#9933=CARTESIAN_POINT('Origin',(0.,0.,16.));
#10220=UNCERTAINTY_MEASURE_WITH_UNIT(LENGTH_MEASURE(0.001),#10266,
'DISTANCE_ACCURACY_VALUE',
'Maximum model space distance between geometric entities at asserted c
onnectivities');
#10227=UNCERTAINTY_MEASURE_WITH_UNIT(LENGTH_MEASURE(0.001),#10266,
'DISTANCE_ACCURACY_VALUE',
'Maximum model space distance between geometric entities at asserted c
onnectivities');
#10258=(
GEOMETRIC_REPRESENTATION_CONTEXT(3)
GLOBAL_UNCERTAINTY_ASSIGNED_CONTEXT((#10220))
GLOBAL_UNIT_ASSIGNED_CONTEXT((#10266,#10268,#10269))
REPRESENTATION_CONTEXT('','3D')
);
#10265=(
GEOMETRIC_REPRESENTATION_CONTEXT(3)
GLOBAL_UNCERTAINTY_ASSIGNED_CONTEXT((#10227))
GLOBAL_UNIT_ASSIGNED_CONTEXT((#10266,#10268,#10269))
REPRESENTATION_CONTEXT('','3D')
);
#10266=(
LENGTH_UNIT()
NAMED_UNIT(*)
SI_UNIT(.CENTI.,.METRE.)
);
#10268=(
NAMED_UNIT(*)
PLANE_ANGLE_UNIT()
SI_UNIT($,.RADIAN.)
);
#10269=(
NAMED_UNIT(*)
SI_UNIT($,.STERADIAN.)
SOLID_ANGLE_UNIT()
);
#10300=SHAPE_DEFINITION_REPRESENTATION(#10341,#10434);
#10341=PRODUCT_DEFINITION_SHAPE('',$,#10472);
#10434=SHAPE_REPRESENTATION('',(#5901),#10258);
#10441=PRODUCT_DEFINITION_CONTEXT('part definition',#10554,'design');
#10472=PRODUCT_DEFINITION('Stop blade','Stop blade',#10509,#10441);
#10509=PRODUCT_DEFINITION_FORMATION('',$,#10586);
#10554=APPLICATION_CONTEXT(
'Core Data for Automotive Mechanical Design Process');
#10555=PRODUCT_CONTEXT('part definition',#10554,'mechanical');
#10586=PRODUCT('Stop blade','Stop blade','Stop blade',(#10555));
#10635=COLOUR_RGB('Light Blue',0.38,0.62,0.78);
#10636=FILL_AREA_STYLE_COLOUR('',#10635);
#10637=FILL_AREA_STYLE('',(#10636));
#10638=SURFACE_STYLE_FILL_AREA(#10637);
#10639=SURFACE_SIDE_STYLE('',(#10638));
#10640=SURFACE_STYLE_USAGE(.BOTH.,#10639);
#10641=PRESENTATION_STYLE_ASSIGNMENT((#10640));
ENDSEC;
END-ISO-10303-21;
